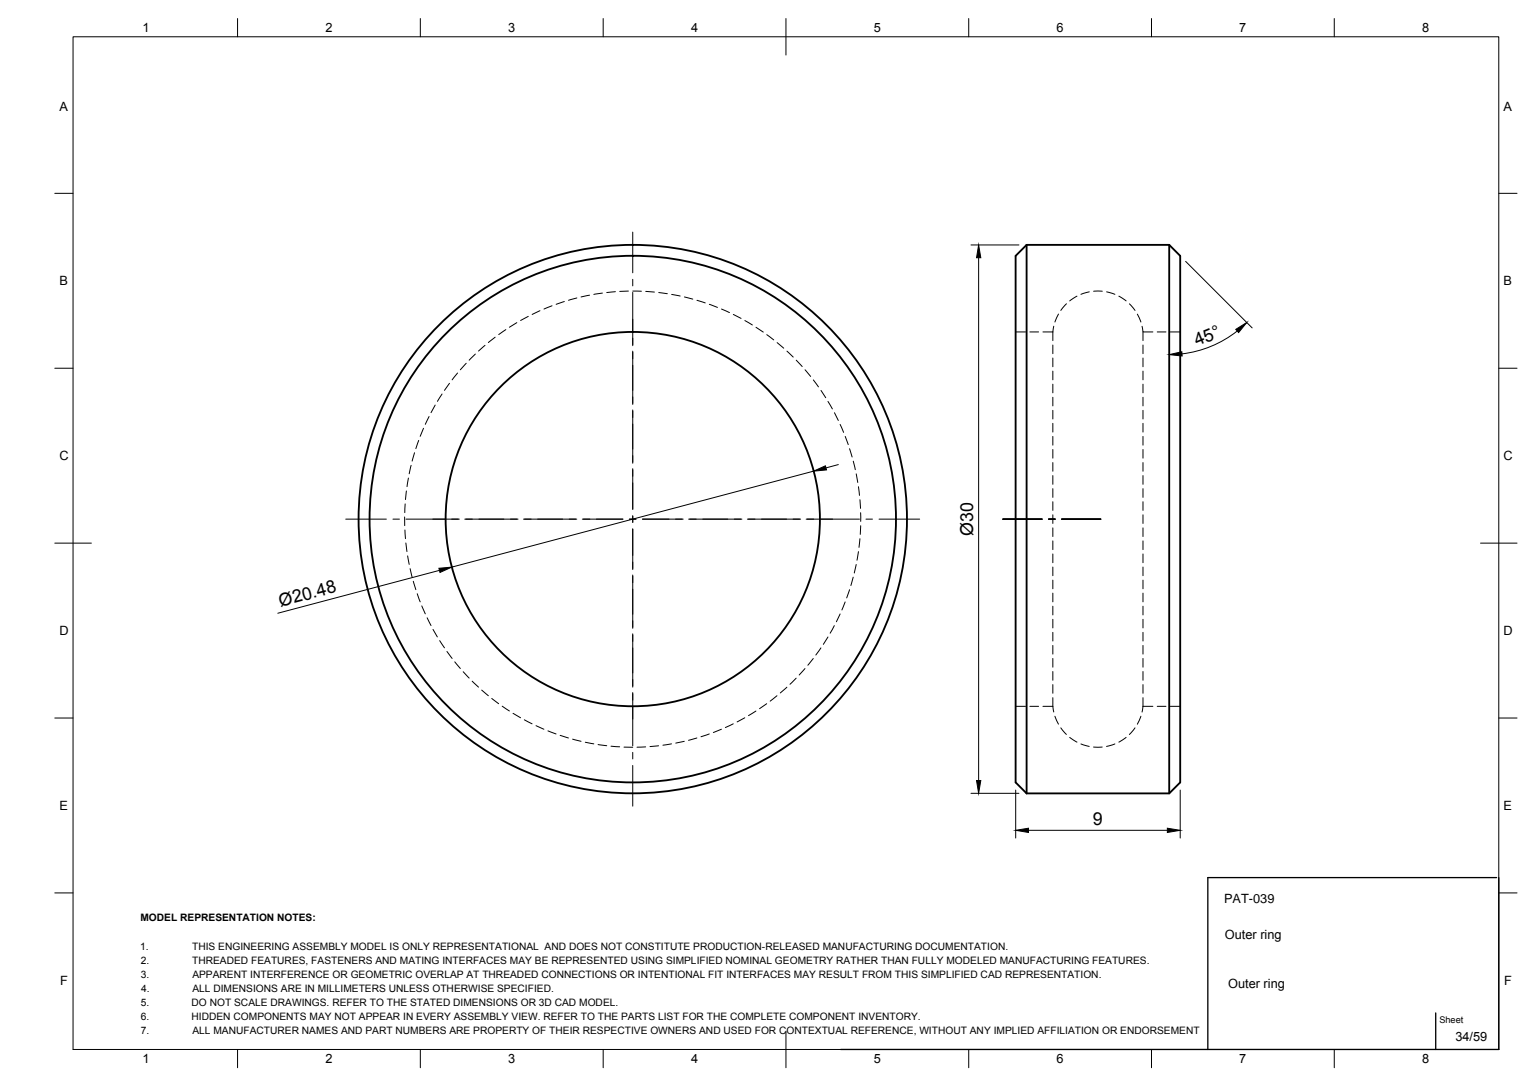
ISO-10303-21;
HEADER;
/* Generated by software containing ST-Developer
 * from STEP Tools, Inc. (www.steptools.com) 
 */

FILE_DESCRIPTION(
/* description */ ('Four-bar parallelogram arm'),
/* implementation_level */ '2;1');

FILE_NAME(
/* name */ 'Outer ring.step',
/* time_stamp */ '2026-10-28T03:24:55-07:00',
/* author */ (''),
/* organization */ (''),
/* preprocessor_version */ 'ST-DEVELOPER v20.2',
/* originating_system */ 'Autodesk Translation Framework v15.17.0.0',
/* authorisation */ '');

FILE_SCHEMA (('AUTOMOTIVE_DESIGN { 1 0 10303 214 3 1 1 }'));
ENDSEC;

DATA;
#10=MECHANICAL_DESIGN_GEOMETRIC_PRESENTATION_REPRESENTATION('',(#655),#14512);
#476=TOROIDAL_SURFACE('',#8528,1.,0.247676);
#482=CONICAL_SURFACE('',#8539,1.47,0.785398163397449);
#483=CONICAL_SURFACE('',#8543,1.47,0.785398163397449);
#555=SHAPE_REPRESENTATION_RELATIONSHIP('SRR','None',#14779,#605);
#605=ADVANCED_BREP_SHAPE_REPRESENTATION('',(#712),#14494);
#655=STYLED_ITEM('',(#15087),#712);
#712=MANIFOLD_SOLID_BREP('Body1',#7360);
#939=FACE_BOUND('',#2095,.T.);
#940=FACE_BOUND('',#2100,.T.);
#1129=PLANE('',#8536);
#1130=PLANE('',#8545);
#1468=FACE_OUTER_BOUND('',#2092,.T.);
#1469=FACE_OUTER_BOUND('',#2093,.T.);
#1470=FACE_OUTER_BOUND('',#2094,.T.);
#1471=FACE_OUTER_BOUND('',#2096,.T.);
#1472=FACE_OUTER_BOUND('',#2097,.T.);
#1473=FACE_OUTER_BOUND('',#2098,.T.);
#1474=FACE_OUTER_BOUND('',#2099,.T.);
#1475=FACE_OUTER_BOUND('',#2101,.T.);
#2092=EDGE_LOOP('',(#6116,#6117,#6118,#6119,#6120,#6121));
#2093=EDGE_LOOP('',(#6122,#6123,#6124,#6125,#6126));
#2094=EDGE_LOOP('',(#6127));
#2095=EDGE_LOOP('',(#6128));
#2096=EDGE_LOOP('',(#6129,#6130,#6131,#6132));
#2097=EDGE_LOOP('',(#6133,#6134,#6135,#6136));
#2098=EDGE_LOOP('',(#6137,#6138,#6139,#6140));
#2099=EDGE_LOOP('',(#6141));
#2100=EDGE_LOOP('',(#6142));
#2101=EDGE_LOOP('',(#6143,#6144,#6145,#6146,#6147));
#2585=LINE('',#13286,#2979);
#2586=LINE('',#13295,#2980);
#2587=LINE('',#13299,#2981);
#2588=LINE('',#13303,#2982);
#2589=LINE('',#13306,#2983);
#2979=VECTOR('',#10439,1.023815);
#2980=VECTOR('',#10450,1.47);
#2981=VECTOR('',#10455,1.5);
#2982=VECTOR('',#10460,1.47);
#2983=VECTOR('',#10465,1.023815);
#3385=CIRCLE('',#8529,1.023815);
#3386=CIRCLE('',#8530,1.023815);
#3387=CIRCLE('',#8531,0.247676);
#3388=CIRCLE('',#8532,1.023815);
#3389=CIRCLE('',#8533,1.023815);
#3390=CIRCLE('',#8535,1.023815);
#3391=CIRCLE('',#8537,1.44);
#3392=CIRCLE('',#8538,1.023815);
#3393=CIRCLE('',#8540,1.5);
#3394=CIRCLE('',#8542,1.5);
#3395=CIRCLE('',#8544,1.44);
#3918=VERTEX_POINT('',#13274);
#3919=VERTEX_POINT('',#13275);
#3920=VERTEX_POINT('',#13278);
#3921=VERTEX_POINT('',#13280);
#3922=VERTEX_POINT('',#13284);
#3923=VERTEX_POINT('',#13288);
#3924=VERTEX_POINT('',#13290);
#3925=VERTEX_POINT('',#13293);
#3926=VERTEX_POINT('',#13297);
#3927=VERTEX_POINT('',#13301);
#4689=EDGE_CURVE('',#3918,#3919,#3385,.T.);
#4690=EDGE_CURVE('',#3919,#3918,#3386,.T.);
#4691=EDGE_CURVE('',#3919,#3920,#3387,.T.);
#4692=EDGE_CURVE('',#3921,#3920,#3388,.T.);
#4693=EDGE_CURVE('',#3920,#3921,#3389,.T.);
#4694=EDGE_CURVE('',#3922,#3922,#3390,.T.);
#4695=EDGE_CURVE('',#3922,#3921,#2585,.T.);
#4696=EDGE_CURVE('',#3923,#3923,#3391,.T.);
#4697=EDGE_CURVE('',#3924,#3924,#3392,.T.);
#4698=EDGE_CURVE('',#3925,#3925,#3393,.T.);
#4699=EDGE_CURVE('',#3925,#3923,#2586,.T.);
#4700=EDGE_CURVE('',#3926,#3926,#3394,.T.);
#4701=EDGE_CURVE('',#3926,#3925,#2587,.T.);
#4702=EDGE_CURVE('',#3927,#3927,#3395,.T.);
#4703=EDGE_CURVE('',#3927,#3926,#2588,.T.);
#4704=EDGE_CURVE('',#3918,#3924,#2589,.T.);
#6116=ORIENTED_EDGE('',*,*,#4689,.F.);
#6117=ORIENTED_EDGE('',*,*,#4690,.F.);
#6118=ORIENTED_EDGE('',*,*,#4691,.T.);
#6119=ORIENTED_EDGE('',*,*,#4692,.F.);
#6120=ORIENTED_EDGE('',*,*,#4693,.F.);
#6121=ORIENTED_EDGE('',*,*,#4691,.F.);
#6122=ORIENTED_EDGE('',*,*,#4694,.T.);
#6123=ORIENTED_EDGE('',*,*,#4695,.T.);
#6124=ORIENTED_EDGE('',*,*,#4692,.T.);
#6125=ORIENTED_EDGE('',*,*,#4693,.T.);
#6126=ORIENTED_EDGE('',*,*,#4695,.F.);
#6127=ORIENTED_EDGE('',*,*,#4696,.F.);
#6128=ORIENTED_EDGE('',*,*,#4697,.T.);
#6129=ORIENTED_EDGE('',*,*,#4698,.F.);
#6130=ORIENTED_EDGE('',*,*,#4699,.T.);
#6131=ORIENTED_EDGE('',*,*,#4696,.T.);
#6132=ORIENTED_EDGE('',*,*,#4699,.F.);
#6133=ORIENTED_EDGE('',*,*,#4700,.F.);
#6134=ORIENTED_EDGE('',*,*,#4701,.T.);
#6135=ORIENTED_EDGE('',*,*,#4698,.T.);
#6136=ORIENTED_EDGE('',*,*,#4701,.F.);
#6137=ORIENTED_EDGE('',*,*,#4702,.F.);
#6138=ORIENTED_EDGE('',*,*,#4703,.T.);
#6139=ORIENTED_EDGE('',*,*,#4700,.T.);
#6140=ORIENTED_EDGE('',*,*,#4703,.F.);
#6141=ORIENTED_EDGE('',*,*,#4702,.T.);
#6142=ORIENTED_EDGE('',*,*,#4694,.F.);
#6143=ORIENTED_EDGE('',*,*,#4689,.T.);
#6144=ORIENTED_EDGE('',*,*,#4690,.T.);
#6145=ORIENTED_EDGE('',*,*,#4704,.T.);
#6146=ORIENTED_EDGE('',*,*,#4697,.F.);
#6147=ORIENTED_EDGE('',*,*,#4704,.F.);
#6851=CYLINDRICAL_SURFACE('',#8534,1.023815);
#6852=CYLINDRICAL_SURFACE('',#8541,1.5);
#6853=CYLINDRICAL_SURFACE('',#8546,1.023815);
#7173=ADVANCED_FACE('',(#1468),#476,.F.);
#7174=ADVANCED_FACE('',(#1469),#6851,.F.);
#7175=ADVANCED_FACE('',(#1470,#939),#1129,.T.);
#7176=ADVANCED_FACE('',(#1471),#482,.T.);
#7177=ADVANCED_FACE('',(#1472),#6852,.T.);
#7178=ADVANCED_FACE('',(#1473),#483,.T.);
#7179=ADVANCED_FACE('',(#1474,#940),#1130,.T.);
#7180=ADVANCED_FACE('',(#1475),#6853,.F.);
#7360=CLOSED_SHELL('',(#7173,#7174,#7175,#7176,#7177,#7178,#7179,#7180));
#8527=AXIS2_PLACEMENT_3D('',#13272,#10421,#10422);
#8528=AXIS2_PLACEMENT_3D('',#13273,#10423,#10424);
#8529=AXIS2_PLACEMENT_3D('',#13276,#10425,#10426);
#8530=AXIS2_PLACEMENT_3D('',#13277,#10427,#10428);
#8531=AXIS2_PLACEMENT_3D('',#13279,#10429,#10430);
#8532=AXIS2_PLACEMENT_3D('',#13281,#10431,#10432);
#8533=AXIS2_PLACEMENT_3D('',#13282,#10433,#10434);
#8534=AXIS2_PLACEMENT_3D('',#13283,#10435,#10436);
#8535=AXIS2_PLACEMENT_3D('',#13285,#10437,#10438);
#8536=AXIS2_PLACEMENT_3D('',#13287,#10440,#10441);
#8537=AXIS2_PLACEMENT_3D('',#13289,#10442,#10443);
#8538=AXIS2_PLACEMENT_3D('',#13291,#10444,#10445);
#8539=AXIS2_PLACEMENT_3D('',#13292,#10446,#10447);
#8540=AXIS2_PLACEMENT_3D('',#13294,#10448,#10449);
#8541=AXIS2_PLACEMENT_3D('',#13296,#10451,#10452);
#8542=AXIS2_PLACEMENT_3D('',#13298,#10453,#10454);
#8543=AXIS2_PLACEMENT_3D('',#13300,#10456,#10457);
#8544=AXIS2_PLACEMENT_3D('',#13302,#10458,#10459);
#8545=AXIS2_PLACEMENT_3D('',#13304,#10461,#10462);
#8546=AXIS2_PLACEMENT_3D('',#13305,#10463,#10464);
#10421=DIRECTION('axis',(0.,0.,1.));
#10422=DIRECTION('refdir',(1.,0.,0.));
#10423=DIRECTION('center_axis',(0.,-1.,0.));
#10424=DIRECTION('ref_axis',(0.,0.,-1.));
#10425=DIRECTION('center_axis',(0.,-1.,0.));
#10426=DIRECTION('ref_axis',(1.,0.,0.));
#10427=DIRECTION('center_axis',(0.,-1.,0.));
#10428=DIRECTION('ref_axis',(1.,0.,0.));
#10429=DIRECTION('center_axis',(1.,0.,1.22464679914735E-16));
#10430=DIRECTION('ref_axis',(-1.22464679914735E-16,0.,1.));
#10431=DIRECTION('center_axis',(0.,1.,0.));
#10432=DIRECTION('ref_axis',(1.,0.,0.));
#10433=DIRECTION('center_axis',(0.,1.,0.));
#10434=DIRECTION('ref_axis',(1.,0.,0.));
#10435=DIRECTION('center_axis',(0.,-1.,0.));
#10436=DIRECTION('ref_axis',(1.,0.,0.));
#10437=DIRECTION('center_axis',(0.,-1.,0.));
#10438=DIRECTION('ref_axis',(1.,0.,0.));
#10439=DIRECTION('',(0.,1.,0.));
#10440=DIRECTION('center_axis',(0.,1.,0.));
#10441=DIRECTION('ref_axis',(0.,0.,1.));
#10442=DIRECTION('center_axis',(0.,-1.,0.));
#10443=DIRECTION('ref_axis',(1.,0.,0.));
#10444=DIRECTION('center_axis',(0.,-1.,0.));
#10445=DIRECTION('ref_axis',(1.,0.,0.));
#10446=DIRECTION('center_axis',(0.,-1.,0.));
#10447=DIRECTION('ref_axis',(1.,0.,0.));
#10448=DIRECTION('center_axis',(0.,-1.,0.));
#10449=DIRECTION('ref_axis',(1.,0.,0.));
#10450=DIRECTION('',(0.707106781186548,0.707106781186547,8.65956056235494E-17));
#10451=DIRECTION('center_axis',(0.,-1.,0.));
#10452=DIRECTION('ref_axis',(1.,0.,0.));
#10453=DIRECTION('center_axis',(0.,-1.,0.));
#10454=DIRECTION('ref_axis',(1.,0.,0.));
#10455=DIRECTION('',(0.,1.,0.));
#10456=DIRECTION('center_axis',(0.,1.,0.));
#10457=DIRECTION('ref_axis',(1.,0.,0.));
#10458=DIRECTION('center_axis',(0.,-1.,0.));
#10459=DIRECTION('ref_axis',(1.,0.,0.));
#10460=DIRECTION('',(-0.707106781186548,0.707106781186547,-8.65956056235494E-17));
#10461=DIRECTION('center_axis',(0.,-1.,0.));
#10462=DIRECTION('ref_axis',(0.,0.,-1.));
#10463=DIRECTION('center_axis',(0.,-1.,0.));
#10464=DIRECTION('ref_axis',(1.,0.,0.));
#10465=DIRECTION('',(0.,1.,0.));
#13272=CARTESIAN_POINT('',(0.,0.,0.));
#13273=CARTESIAN_POINT('Origin',(0.,0.,0.));
#13274=CARTESIAN_POINT('',(-1.023815,0.246528389340863,-1.25381176266905E-16));
#13275=CARTESIAN_POINT('',(-1.25381176266905E-16,0.246528389340863,1.023815));
#13276=CARTESIAN_POINT('Origin',(0.,0.246528389340863,0.));
#13277=CARTESIAN_POINT('Origin',(0.,0.246528389340863,0.));
#13278=CARTESIAN_POINT('',(-1.25381176266905E-16,-0.246528389340863,1.023815));
#13279=CARTESIAN_POINT('Origin',(-1.22464679914735E-16,0.,1.));
#13280=CARTESIAN_POINT('',(-1.023815,-0.246528389340863,1.25381176266905E-16));
#13281=CARTESIAN_POINT('Origin',(0.,-0.246528389340863,0.));
#13282=CARTESIAN_POINT('Origin',(0.,-0.246528389340863,0.));
#13283=CARTESIAN_POINT('Origin',(0.,0.,0.));
#13284=CARTESIAN_POINT('',(-1.023815,-0.45,-1.25381176266905E-16));
#13285=CARTESIAN_POINT('Origin',(0.,-0.45,0.));
#13286=CARTESIAN_POINT('',(-1.023815,0.,-1.25381176266905E-16));
#13287=CARTESIAN_POINT('Origin',(1.44,0.45,0.));
#13288=CARTESIAN_POINT('',(-1.44,0.45,-1.76349139077219E-16));
#13289=CARTESIAN_POINT('Origin',(0.,0.45,0.));
#13290=CARTESIAN_POINT('',(-1.023815,0.45,-1.25381176266905E-16));
#13291=CARTESIAN_POINT('Origin',(0.,0.45,0.));
#13292=CARTESIAN_POINT('Origin',(0.,0.42,0.));
#13293=CARTESIAN_POINT('',(-1.5,0.39,-1.83697019872103E-16));
#13294=CARTESIAN_POINT('Origin',(0.,0.39,0.));
#13295=CARTESIAN_POINT('',(-1.47,0.42,-1.80023079474661E-16));
#13296=CARTESIAN_POINT('Origin',(0.,0.,0.));
#13297=CARTESIAN_POINT('',(-1.5,-0.39,-1.83697019872103E-16));
#13298=CARTESIAN_POINT('Origin',(0.,-0.39,0.));
#13299=CARTESIAN_POINT('',(-1.5,0.,-1.83697019872103E-16));
#13300=CARTESIAN_POINT('Origin',(0.,-0.42,0.));
#13301=CARTESIAN_POINT('',(-1.44,-0.45,-1.76349139077219E-16));
#13302=CARTESIAN_POINT('Origin',(0.,-0.45,0.));
#13303=CARTESIAN_POINT('',(-1.47,-0.42,-1.80023079474661E-16));
#13304=CARTESIAN_POINT('Origin',(1.023815,-0.45,0.));
#13305=CARTESIAN_POINT('Origin',(0.,0.,0.));
#13306=CARTESIAN_POINT('',(-1.023815,0.,-1.25381176266905E-16));
#14437=UNCERTAINTY_MEASURE_WITH_UNIT(LENGTH_MEASURE(0.001),#14513,
'DISTANCE_ACCURACY_VALUE',
'Maximum model space distance between geometric entities at asserted c
onnectivities');
#14455=UNCERTAINTY_MEASURE_WITH_UNIT(LENGTH_MEASURE(0.001),#14513,
'DISTANCE_ACCURACY_VALUE',
'Maximum model space distance between geometric entities at asserted c
onnectivities');
#14494=(
GEOMETRIC_REPRESENTATION_CONTEXT(3)
GLOBAL_UNCERTAINTY_ASSIGNED_CONTEXT((#14437))
GLOBAL_UNIT_ASSIGNED_CONTEXT((#14513,#14515,#14516))
REPRESENTATION_CONTEXT('','3D')
);
#14512=(
GEOMETRIC_REPRESENTATION_CONTEXT(3)
GLOBAL_UNCERTAINTY_ASSIGNED_CONTEXT((#14455))
GLOBAL_UNIT_ASSIGNED_CONTEXT((#14513,#14515,#14516))
REPRESENTATION_CONTEXT('','3D')
);
#14513=(
LENGTH_UNIT()
NAMED_UNIT(*)
SI_UNIT(.CENTI.,.METRE.)
);
#14515=(
NAMED_UNIT(*)
PLANE_ANGLE_UNIT()
SI_UNIT($,.RADIAN.)
);
#14516=(
NAMED_UNIT(*)
SI_UNIT($,.STERADIAN.)
SOLID_ANGLE_UNIT()
);
#14555=SHAPE_DEFINITION_REPRESENTATION(#14611,#14779);
#14611=PRODUCT_DEFINITION_SHAPE('',$,#14836);
#14779=SHAPE_REPRESENTATION('',(#8527),#14494);
#14797=PRODUCT_DEFINITION_CONTEXT('part definition',#14967,'design');
#14836=PRODUCT_DEFINITION('Outer ring','Outer ring',#14892,#14797);
#14892=PRODUCT_DEFINITION_FORMATION('',$,#15007);
#14967=APPLICATION_CONTEXT(
'Core Data for Automotive Mechanical Design Process');
#14968=PRODUCT_CONTEXT('part definition',#14967,'mechanical');
#15007=PRODUCT('Outer ring','Outer ring','Outer ring',(#14968));
#15081=COLOUR_RGB('Grey',0.48,0.52,0.57);
#15082=FILL_AREA_STYLE_COLOUR('',#15081);
#15083=FILL_AREA_STYLE('',(#15082));
#15084=SURFACE_STYLE_FILL_AREA(#15083);
#15085=SURFACE_SIDE_STYLE('',(#15084));
#15086=SURFACE_STYLE_USAGE(.BOTH.,#15085);
#15087=PRESENTATION_STYLE_ASSIGNMENT((#15086));
ENDSEC;
END-ISO-10303-21;
